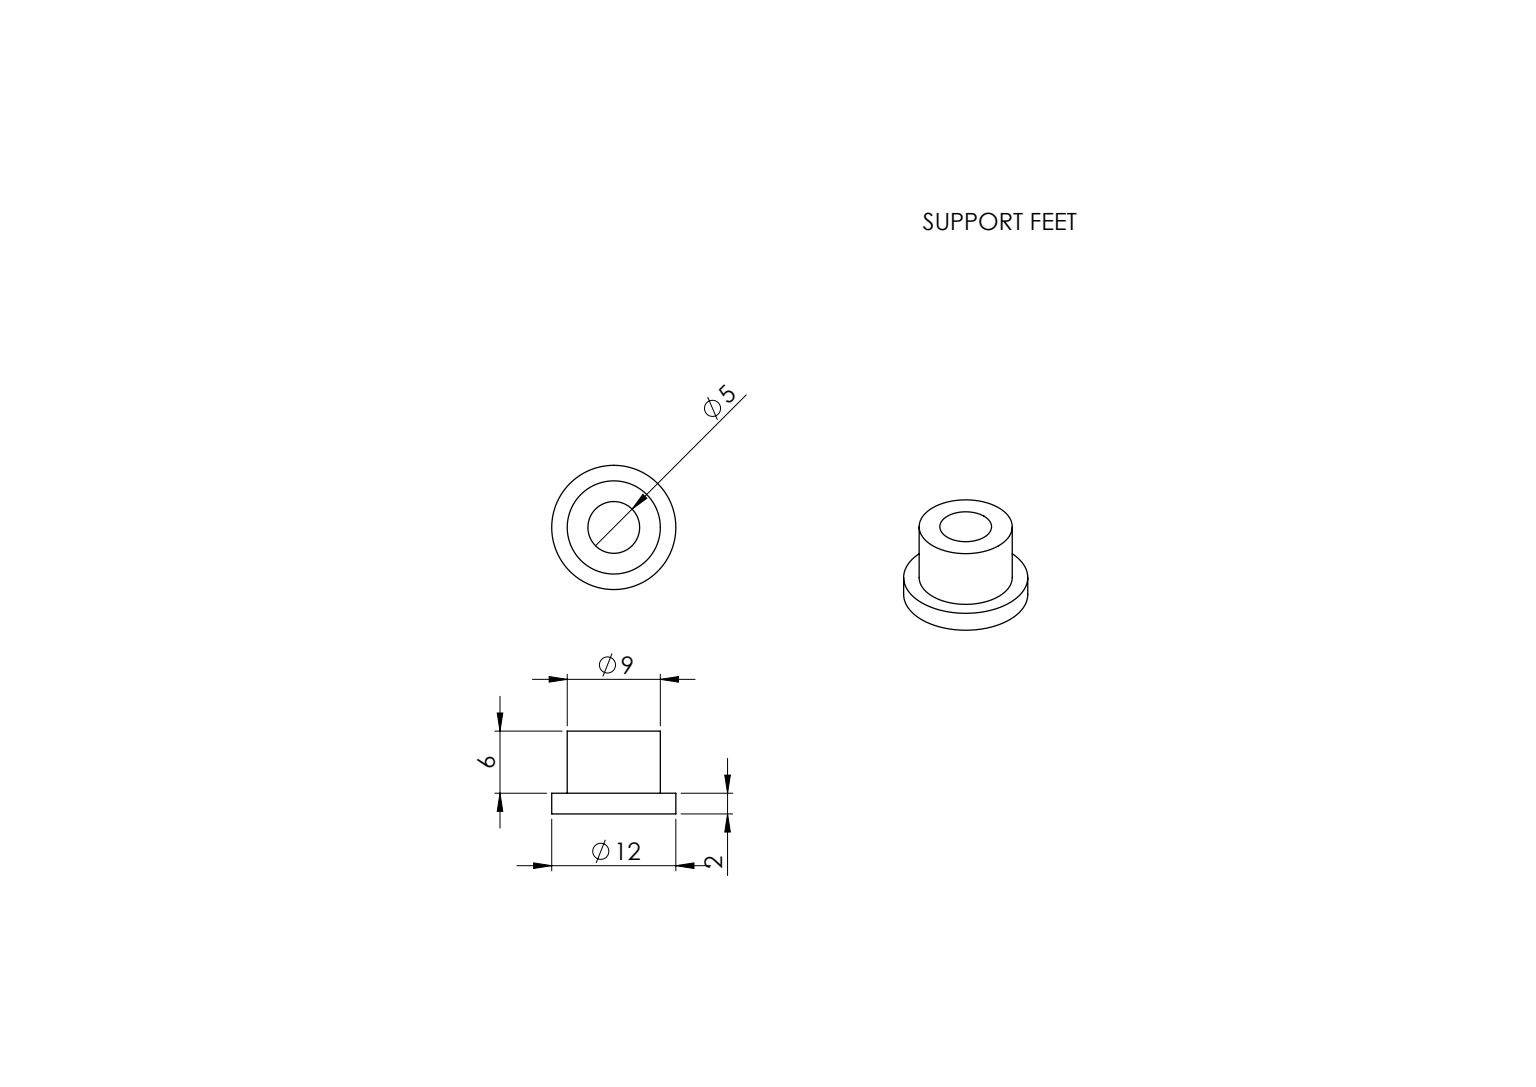
ISO-10303-21;
HEADER;
FILE_DESCRIPTION (('STEP AP214'),
    '1' );
FILE_NAME ('Support Feet^MAS-192.step',
    '2026-10-24T04:45:50',
    ( '' ),
    ( '' ),
    'SwSTEP 2.0',
    'SolidWorks 2026',
    '' );
FILE_SCHEMA (( 'AUTOMOTIVE_DESIGN' ));
ENDSEC;

DATA;
#2=( GEOMETRIC_REPRESENTATION_CONTEXT ( 3 ) GLOBAL_UNCERTAINTY_ASSIGNED_CONTEXT ( ( #2528 ) ) GLOBAL_UNIT_ASSIGNED_CONTEXT ( ( #1633, #2133, #1361 ) ) REPRESENTATION_CONTEXT ( 'NONE', 'WORKASPACE' ) );
#3=DIRECTION ( 'NONE',  ( 0.000000000000000000, -1.000000000000000000, 0.000000000000000000 ) ) ;
#6=ORIENTED_EDGE ( 'NONE', *, *, #1808, .T. ) ;
#13=ORIENTED_EDGE ( 'NONE', *, *, #2082, .F. ) ;
#22=VERTEX_POINT ( 'NONE', #1418 ) ;
#25=PRODUCT ( 'Support Feet^MAS-192', 'Support Feet^MAS-192', '', ( #945 ) ) ;
#74=ORIENTED_EDGE ( 'NONE', *, *, #2863, .T. ) ;
#80=SURFACE_STYLE_USAGE ( .BOTH. , #3231 ) ;
#98=AXIS2_PLACEMENT_3D ( 'NONE', #3255, #906, #600 ) ;
#106=EDGE_CURVE ( 'NONE', #871, #1696, #686, .T. ) ;
#124=ORIENTED_EDGE ( 'NONE', *, *, #674, .T. ) ;
#145=DIRECTION ( 'NONE',  ( -0.000000000000000000, 1.000000000000000000, -0.000000000000000000 ) ) ;
#146=DIRECTION ( 'NONE',  ( 0.000000000000000000, -1.000000000000000000, 0.000000000000000000 ) ) ;
#150=AXIS2_PLACEMENT_3D ( 'NONE', #1095, #3156, #1856 ) ;
#153=MECHANICAL_DESIGN_GEOMETRIC_PRESENTATION_REPRESENTATION('',(#3211),#1787);
#168=ADVANCED_FACE ( 'NONE', ( #219 ), #472, .F. ) ;
#179=SHAPE_REPRESENTATION_RELATIONSHIP ( 'NONE' , 'NONE' ,  #1050, #930 ) ;
#195=EDGE_CURVE ( 'NONE', #2855, #2405, #2542, .T. ) ;
#201=VECTOR ( 'NONE', #2928, 1000.000000000000000 ) ;
#211=DIRECTION ( 'NONE',  ( 0.000000000000000000, -1.000000000000000000, 0.000000000000000000 ) ) ;
#216=( NAMED_UNIT ( * ) PLANE_ANGLE_UNIT ( ) SI_UNIT ( $, .RADIAN. ) );
#219=FACE_OUTER_BOUND ( 'NONE', #3264, .T. ) ;
#222=DIRECTION ( 'NONE',  ( -0.000000000000000000, 1.000000000000000000, -0.000000000000000000 ) ) ;
#245=ORIENTED_EDGE ( 'NONE', *, *, #2920, .T. ) ;
#251=CARTESIAN_POINT ( 'NONE',  ( -66.99999999999997158, -6.000000000000000000, 41.99999999999999289 ) ) ;
#254=ORIENTED_EDGE ( 'NONE', *, *, #2827, .T. ) ;
#261=CARTESIAN_POINT ( 'NONE',  ( -66.99999999999997158, -8.000000000000000000, 41.99999999999999289 ) ) ;
#268=AXIS2_PLACEMENT_3D ( 'NONE', #2067, #1047, #3088 ) ;
#291=CYLINDRICAL_SURFACE ( 'NONE', #701, 4.500000000000010658 ) ;
#322=AXIS2_PLACEMENT_3D ( 'NONE', #1317, #3110, #3142 ) ;
#331=VERTEX_POINT ( 'NONE', #2651 ) ;
#340=ORIENTED_EDGE ( 'NONE', *, *, #1808, .F. ) ;
#348=CARTESIAN_POINT ( 'NONE',  ( -66.99999999999997158, 0.000000000000000000, 46.50000000000000711 ) ) ;
#349=SURFACE_STYLE_FILL_AREA ( #2686 ) ;
#364=( LENGTH_UNIT ( ) NAMED_UNIT ( * ) SI_UNIT ( .MILLI., .METRE. ) );
#370=CIRCLE ( 'NONE', #482, 4.500000000000010658 ) ;
#379=AXIS2_PLACEMENT_3D ( 'NONE', #915, #146, #2518 ) ;
#386=ORIENTED_EDGE ( 'NONE', *, *, #1705, .F. ) ;
#388=DIRECTION ( 'NONE',  ( 0.000000000000000000, 0.000000000000000000, -1.000000000000000000 ) ) ;
#405=CARTESIAN_POINT ( 'NONE',  ( -66.99999999999997158, -8.000000000000000000, 39.49999999999998579 ) ) ;
#415=ORIENTED_EDGE ( 'NONE', *, *, #2685, .T. ) ;
#422=CIRCLE ( 'NONE', #2330, 2.500000000000009326 ) ;
#472=CYLINDRICAL_SURFACE ( 'NONE', #803, 2.500000000000009326 ) ;
#482=AXIS2_PLACEMENT_3D ( 'NONE', #711, #2825, #1752 ) ;
#484=CIRCLE ( 'NONE', #975, 6.000000000000005329 ) ;
#506=EDGE_LOOP ( 'NONE', ( #2297, #1009 ) ) ;
#508=CARTESIAN_POINT ( 'NONE',  ( -66.99999999999997158, -8.000000000000000000, 41.99999999999999289 ) ) ;
#513=EDGE_LOOP ( 'NONE', ( #1170, #1121 ) ) ;
#525=ORIENTED_EDGE ( 'NONE', *, *, #1492, .F. ) ;
#535=EDGE_CURVE ( 'NONE', #871, #3340, #2736, .T. ) ;
#536=AXIS2_PLACEMENT_3D ( 'NONE', #3344, #1291, #2041 ) ;
#547=ORIENTED_EDGE ( 'NONE', *, *, #1705, .T. ) ;
#589=CIRCLE ( 'NONE', #1031, 4.500000000000010658 ) ;
#593=CIRCLE ( 'NONE', #268, 6.000000000000005329 ) ;
#596=ADVANCED_FACE ( 'NONE', ( #3051 ), #1293, .T. ) ;
#600=DIRECTION ( 'NONE',  ( 0.000000000000000000, 0.000000000000000000, -1.000000000000000000 ) ) ;
#606=CARTESIAN_POINT ( 'NONE',  ( -66.99999999999997158, -6.000000000000000000, 44.50000000000000711 ) ) ;
#617=VERTEX_POINT ( 'NONE', #1508 ) ;
#637=AXIS2_PLACEMENT_3D ( 'NONE', #2080, #3362, #966 ) ;
#650=CARTESIAN_POINT ( 'NONE',  ( -66.99999999999997158, 0.000000000000000000, 41.99999999999999289 ) ) ;
#662=CYLINDRICAL_SURFACE ( 'NONE', #1528, 6.000000000000005329 ) ;
#665=DIRECTION ( 'NONE',  ( 0.000000000000000000, -0.000000000000000000, -1.000000000000000000 ) ) ;
#666=EDGE_CURVE ( 'NONE', #617, #22, #2260, .T. ) ;
#674=EDGE_CURVE ( 'NONE', #2405, #2855, #370, .T. ) ;
#681=SHAPE_DEFINITION_REPRESENTATION ( #1034, #1050 ) ;
#686=CIRCLE ( 'NONE', #858, 2.500000000000009326 ) ;
#701=AXIS2_PLACEMENT_3D ( 'NONE', #1590, #222, #1270 ) ;
#711=CARTESIAN_POINT ( 'NONE',  ( -66.99999999999997158, -6.000000000000000000, 41.99999999999999289 ) ) ;
#725=UNCERTAINTY_MEASURE_WITH_UNIT (LENGTH_MEASURE( 1.000000000000000082E-05 ), #364, 'distance_accuracy_value', 'NONE');
#744=DIRECTION ( 'NONE',  ( 0.000000000000000000, -0.000000000000000000, -1.000000000000000000 ) ) ;
#753=FACE_OUTER_BOUND ( 'NONE', #969, .T. ) ;
#760=UNCERTAINTY_MEASURE_WITH_UNIT (LENGTH_MEASURE( 1.000000000000000082E-05 ), #1279, 'distance_accuracy_value', 'NONE');
#767=EDGE_CURVE ( 'NONE', #3340, #1840, #1842, .T. ) ;
#778=ORIENTED_EDGE ( 'NONE', *, *, #535, .T. ) ;
#799=CARTESIAN_POINT ( 'NONE',  ( -66.99999999999997158, -6.000000000000000000, 48.00000000000000000 ) ) ;
#803=AXIS2_PLACEMENT_3D ( 'NONE', #508, #1247, #1756 ) ;
#853=CARTESIAN_POINT ( 'NONE',  ( -66.99999999999997158, -6.000000000000000000, 41.99999999999999289 ) ) ;
#858=AXIS2_PLACEMENT_3D ( 'NONE', #3313, #2011, #3055 ) ;
#871=VERTEX_POINT ( 'NONE', #929 ) ;
#877=EDGE_LOOP ( 'NONE', ( #13, #2657 ) ) ;
#882=PRESENTATION_STYLE_ASSIGNMENT (( #80 ) ) ;
#906=DIRECTION ( 'NONE',  ( 0.000000000000000000, -1.000000000000000000, 0.000000000000000000 ) ) ;
#909=CARTESIAN_POINT ( 'NONE',  ( -66.99999999999997158, 0.000000000000000000, 41.99999999999999289 ) ) ;
#915=CARTESIAN_POINT ( 'NONE',  ( -66.99999999999997158, -6.000000000000000000, 41.99999999999999289 ) ) ;
#925=VECTOR ( 'NONE', #3, 1000.000000000000000 ) ;
#929=CARTESIAN_POINT ( 'NONE',  ( -66.99999999999997158, -6.000000000000000000, 39.49999999999998579 ) ) ;
#930=ADVANCED_BREP_SHAPE_REPRESENTATION ( '', ( #2021, #3111 ), #2 ) ;
#938=CARTESIAN_POINT ( 'NONE',  ( -66.99999999999997158, -8.000000000000000000, 44.50000000000000711 ) ) ;
#945=PRODUCT_CONTEXT ( 'NONE', #1857, 'mechanical' ) ;
#966=DIRECTION ( 'NONE',  ( 0.000000000000000000, 0.000000000000000000, -1.000000000000000000 ) ) ;
#969=EDGE_LOOP ( 'NONE', ( #2568, #3228 ) ) ;
#974=CARTESIAN_POINT ( 'NONE',  ( -66.99999999999997158, -6.000000000000000000, 48.00000000000000000 ) ) ;
#975=AXIS2_PLACEMENT_3D ( 'NONE', #261, #211, #2079 ) ;
#1002=CARTESIAN_POINT ( 'NONE',  ( -66.99999999999997158, -6.000000000000000000, 35.99999999999999289 ) ) ;
#1005=FACE_BOUND ( 'NONE', #506, .T. ) ;
#1009=ORIENTED_EDGE ( 'NONE', *, *, #767, .T. ) ;
#1014=ADVANCED_FACE ( 'NONE', ( #753 ), #1776, .F. ) ;
#1031=AXIS2_PLACEMENT_3D ( 'NONE', #650, #1156, #1434 ) ;
#1034=PRODUCT_DEFINITION_SHAPE ( 'NONE', 'NONE',  #2584 ) ;
#1047=DIRECTION ( 'NONE',  ( 0.000000000000000000, -1.000000000000000000, 0.000000000000000000 ) ) ;
#1050=SHAPE_REPRESENTATION ( 'Support Feet^MAS-192', ( #3111 ), #2 ) ;
#1084=AXIS2_PLACEMENT_3D ( 'NONE', #251, #2301, #2316 ) ;
#1090=AXIS2_PLACEMENT_3D ( 'NONE', #2616, #2119, #3356 ) ;
#1095=CARTESIAN_POINT ( 'NONE',  ( -66.99999999999997158, 0.000000000000000000, 41.99999999999999289 ) ) ;
#1121=ORIENTED_EDGE ( 'NONE', *, *, #1492, .T. ) ;
#1138=ORIENTED_EDGE ( 'NONE', *, *, #1885, .T. ) ;
#1145=AXIS2_PLACEMENT_3D ( 'NONE', #853, #2462, #1878 ) ;
#1156=DIRECTION ( 'NONE',  ( 0.000000000000000000, -1.000000000000000000, 0.000000000000000000 ) ) ;
#1170=ORIENTED_EDGE ( 'NONE', *, *, #2436, .T. ) ;
#1171=ADVANCED_FACE ( 'NONE', ( #2692, #2203 ), #3199, .F. ) ;
#1196=FACE_OUTER_BOUND ( 'NONE', #2237, .T. ) ;
#1208=MECHANICAL_DESIGN_GEOMETRIC_PRESENTATION_REPRESENTATION('',(#1468),#3054);
#1209=ORIENTED_EDGE ( 'NONE', *, *, #666, .T. ) ;
#1215=DIRECTION ( 'NONE',  ( -0.000000000000000000, 1.000000000000000000, -0.000000000000000000 ) ) ;
#1224=ORIENTED_EDGE ( 'NONE', *, *, #2353, .F. ) ;
#1229=CARTESIAN_POINT ( 'NONE',  ( -66.99999999999997158, 0.000000000000000000, 44.50000000000000711 ) ) ;
#1244=CIRCLE ( 'NONE', #379, 2.500000000000009326 ) ;
#1247=DIRECTION ( 'NONE',  ( -0.000000000000000000, 1.000000000000000000, -0.000000000000000000 ) ) ;
#1262=CARTESIAN_POINT ( 'NONE',  ( -66.99999999999997158, -6.000000000000000000, 37.49999999999998579 ) ) ;
#1270=DIRECTION ( 'NONE',  ( 0.000000000000000000, 0.000000000000000000, 1.000000000000000000 ) ) ;
#1279=( LENGTH_UNIT ( ) NAMED_UNIT ( * ) SI_UNIT ( .MILLI., .METRE. ) );
#1291=DIRECTION ( 'NONE',  ( -0.000000000000000000, 1.000000000000000000, -0.000000000000000000 ) ) ;
#1293=CYLINDRICAL_SURFACE ( 'NONE', #637, 6.000000000000005329 ) ;
#1314=CARTESIAN_POINT ( 'NONE',  ( -66.99999999999997158, 0.000000000000000000, 37.49999999999998579 ) ) ;
#1317=CARTESIAN_POINT ( 'NONE',  ( -66.99999999999997158, -8.000000000000000000, 41.99999999999999289 ) ) ;
#1361=( NAMED_UNIT ( * ) SI_UNIT ( $, .STERADIAN. ) SOLID_ANGLE_UNIT ( ) );
#1394=CYLINDRICAL_SURFACE ( 'NONE', #3329, 4.500000000000010658 ) ;
#1418=CARTESIAN_POINT ( 'NONE',  ( -66.99999999999997158, -8.000000000000000000, 35.99999999999999289 ) ) ;
#1432=ORIENTED_EDGE ( 'NONE', *, *, #2774, .F. ) ;
#1434=DIRECTION ( 'NONE',  ( 1.000000000000000000, 0.000000000000000000, 0.000000000000000000 ) ) ;
#1464=VECTOR ( 'NONE', #2850, 1000.000000000000000 ) ;
#1468=STYLED_ITEM ( 'NONE', ( #882 ), #930 ) ;
#1470=COLOUR_RGB ( '',0.8941176470588234615, 0.8941176470588234615, 0.8941176470588234615 ) ;
#1492=EDGE_CURVE ( 'NONE', #331, #22, #2340, .T. ) ;
#1508=CARTESIAN_POINT ( 'NONE',  ( -66.99999999999997158, -6.000000000000000000, 35.99999999999999289 ) ) ;
#1528=AXIS2_PLACEMENT_3D ( 'NONE', #2778, #3031, #2008 ) ;
#1575=CIRCLE ( 'NONE', #2713, 6.000000000000005329 ) ;
#1579=AXIS2_PLACEMENT_3D ( 'NONE', #1963, #2758, #665 ) ;
#1590=CARTESIAN_POINT ( 'NONE',  ( -66.99999999999997158, -8.000000000000000000, 41.99999999999999289 ) ) ;
#1591=EDGE_LOOP ( 'NONE', ( #2711, #1432 ) ) ;
#1603=CARTESIAN_POINT ( 'NONE',  ( -66.99999999999997158, -8.000000000000000000, 41.99999999999999289 ) ) ;
#1633=( LENGTH_UNIT ( ) NAMED_UNIT ( * ) SI_UNIT ( .MILLI., .METRE. ) );
#1696=VERTEX_POINT ( 'NONE', #606 ) ;
#1705=EDGE_CURVE ( 'NONE', #2405, #2003, #2149, .T. ) ;
#1723=PLANE ( 'NONE',  #1579 ) ;
#1752=DIRECTION ( 'NONE',  ( 0.000000000000000000, 0.000000000000000000, -1.000000000000000000 ) ) ;
#1756=DIRECTION ( 'NONE',  ( 0.000000000000000000, 0.000000000000000000, 1.000000000000000000 ) ) ;
#1776=PLANE ( 'NONE',  #1090 ) ;
#1787=( GEOMETRIC_REPRESENTATION_CONTEXT ( 3 ) GLOBAL_UNCERTAINTY_ASSIGNED_CONTEXT ( ( #760 ) ) GLOBAL_UNIT_ASSIGNED_CONTEXT ( ( #1279, #216, #2094 ) ) REPRESENTATION_CONTEXT ( 'NONE', 'WORKASPACE' ) );
#1808=EDGE_CURVE ( 'NONE', #1696, #1840, #1986, .T. ) ;
#1809=CARTESIAN_POINT ( 'NONE',  ( -66.99999999999997158, -6.000000000000000000, 46.50000000000000711 ) ) ;
#1838=VECTOR ( 'NONE', #145, 1000.000000000000000 ) ;
#1840=VERTEX_POINT ( 'NONE', #1229 ) ;
#1842=CIRCLE ( 'NONE', #98, 2.500000000000009326 ) ;
#1856=DIRECTION ( 'NONE',  ( 1.000000000000000000, 0.000000000000000000, 0.000000000000000000 ) ) ;
#1857=APPLICATION_CONTEXT ( 'automotive_design' ) ;
#1861=CARTESIAN_POINT ( 'NONE',  ( -66.99999999999997158, -8.000000000000000000, 46.50000000000000711 ) ) ;
#1871=CARTESIAN_POINT ( 'NONE',  ( 0.000000000000000000, 0.000000000000000000, 0.000000000000000000 ) ) ;
#1878=DIRECTION ( 'NONE',  ( 0.000000000000000000, -0.000000000000000000, -1.000000000000000000 ) ) ;
#1885=EDGE_CURVE ( 'NONE', #1696, #871, #1244, .T. ) ;
#1938=DIRECTION ( 'NONE',  ( 0.000000000000000000, 0.000000000000000000, 1.000000000000000000 ) ) ;
#1963=CARTESIAN_POINT ( 'NONE',  ( -66.99999999999997158, -8.000000000000000000, 41.99999999999999289 ) ) ;
#1978=LINE ( 'NONE', #1861, #1464 ) ;
#1986=LINE ( 'NONE', #938, #3167 ) ;
#1993=CARTESIAN_POINT ( 'NONE',  ( -66.99999999999997158, -6.000000000000000000, 41.99999999999999289 ) ) ;
#2003=VERTEX_POINT ( 'NONE', #1314 ) ;
#2008=DIRECTION ( 'NONE',  ( 0.000000000000000000, 0.000000000000000000, -1.000000000000000000 ) ) ;
#2011=DIRECTION ( 'NONE',  ( 0.000000000000000000, -1.000000000000000000, 0.000000000000000000 ) ) ;
#2014=FACE_OUTER_BOUND ( 'NONE', #513, .T. ) ;
#2021=MANIFOLD_SOLID_BREP ( 'Boss-Extrude1', #2700 ) ;
#2041=DIRECTION ( 'NONE',  ( 0.000000000000000000, 0.000000000000000000, 1.000000000000000000 ) ) ;
#2049=EDGE_LOOP ( 'NONE', ( #2469, #124 ) ) ;
#2057=ORIENTED_EDGE ( 'NONE', *, *, #2082, .T. ) ;
#2067=CARTESIAN_POINT ( 'NONE',  ( -66.99999999999997158, -6.000000000000000000, 41.99999999999999289 ) ) ;
#2079=DIRECTION ( 'NONE',  ( 0.000000000000000000, 0.000000000000000000, -1.000000000000000000 ) ) ;
#2080=CARTESIAN_POINT ( 'NONE',  ( -66.99999999999997158, -6.000000000000000000, 41.99999999999999289 ) ) ;
#2082=EDGE_CURVE ( 'NONE', #2103, #2003, #2988, .T. ) ;
#2094=( NAMED_UNIT ( * ) SI_UNIT ( $, .STERADIAN. ) SOLID_ANGLE_UNIT ( ) );
#2103=VERTEX_POINT ( 'NONE', #348 ) ;
#2117=VECTOR ( 'NONE', #3309, 1000.000000000000000 ) ;
#2119=DIRECTION ( 'NONE',  ( 0.000000000000000000, -1.000000000000000000, 0.000000000000000000 ) ) ;
#2133=( NAMED_UNIT ( * ) PLANE_ANGLE_UNIT ( ) SI_UNIT ( $, .RADIAN. ) );
#2147=FILL_AREA_STYLE_COLOUR ( '', #1470 ) ;
#2149=LINE ( 'NONE', #2383, #201 ) ;
#2150=FACE_OUTER_BOUND ( 'NONE', #2581, .T. ) ;
#2159=ORIENTED_EDGE ( 'NONE', *, *, #535, .F. ) ;
#2203=FACE_OUTER_BOUND ( 'NONE', #1591, .T. ) ;
#2216=DIRECTION ( 'NONE',  ( 0.000000000000000000, 0.000000000000000000, -1.000000000000000000 ) ) ;
#2237=EDGE_LOOP ( 'NONE', ( #74, #245, #2450, #2549 ) ) ;
#2260=LINE ( 'NONE', #1002, #2117 ) ;
#2297=ORIENTED_EDGE ( 'NONE', *, *, #2353, .T. ) ;
#2301=DIRECTION ( 'NONE',  ( 0.000000000000000000, -1.000000000000000000, 0.000000000000000000 ) ) ;
#2316=DIRECTION ( 'NONE',  ( 0.000000000000000000, 0.000000000000000000, -1.000000000000000000 ) ) ;
#2330=AXIS2_PLACEMENT_3D ( 'NONE', #909, #2749, #388 ) ;
#2338=FACE_OUTER_BOUND ( 'NONE', #3118, .T. ) ;
#2340=CIRCLE ( 'NONE', #322, 6.000000000000005329 ) ;
#2349=ORIENTED_EDGE ( 'NONE', *, *, #767, .F. ) ;
#2353=EDGE_CURVE ( 'NONE', #1840, #3340, #422, .T. ) ;
#2354=DIRECTION ( 'NONE',  ( 0.000000000000000000, -1.000000000000000000, 0.000000000000000000 ) ) ;
#2383=CARTESIAN_POINT ( 'NONE',  ( -66.99999999999997158, -8.000000000000000000, 37.49999999999998579 ) ) ;
#2405=VERTEX_POINT ( 'NONE', #1262 ) ;
#2434=DIRECTION ( 'NONE',  ( -0.000000000000000000, 1.000000000000000000, -0.000000000000000000 ) ) ;
#2436=EDGE_CURVE ( 'NONE', #22, #331, #484, .T. ) ;
#2450=ORIENTED_EDGE ( 'NONE', *, *, #2436, .F. ) ;
#2454=( NAMED_UNIT ( * ) PLANE_ANGLE_UNIT ( ) SI_UNIT ( $, .RADIAN. ) );
#2462=DIRECTION ( 'NONE',  ( 0.000000000000000000, -1.000000000000000000, 0.000000000000000000 ) ) ;
#2467=ADVANCED_FACE ( 'NONE', ( #2570 ), #2841, .F. ) ;
#2469=ORIENTED_EDGE ( 'NONE', *, *, #195, .T. ) ;
#2518=DIRECTION ( 'NONE',  ( 0.000000000000000000, 0.000000000000000000, -1.000000000000000000 ) ) ;
#2528=UNCERTAINTY_MEASURE_WITH_UNIT (LENGTH_MEASURE( 1.000000000000000082E-05 ), #1633, 'distance_accuracy_value', 'NONE');
#2542=CIRCLE ( 'NONE', #1084, 4.500000000000010658 ) ;
#2549=ORIENTED_EDGE ( 'NONE', *, *, #666, .F. ) ;
#2568=ORIENTED_EDGE ( 'NONE', *, *, #1885, .F. ) ;
#2570=FACE_OUTER_BOUND ( 'NONE', #3145, .T. ) ;
#2572=PLANE ( 'NONE',  #3278 ) ;
#2581=EDGE_LOOP ( 'NONE', ( #3146, #547, #415, #2890 ) ) ;
#2584=PRODUCT_DEFINITION ( 'UNKNOWN', '', #3229, #3288 ) ;
#2616=CARTESIAN_POINT ( 'NONE',  ( -66.99999999999997158, -6.000000000000000000, 41.99999999999999289 ) ) ;
#2634=ORIENTED_EDGE ( 'NONE', *, *, #106, .T. ) ;
#2639=DIRECTION ( 'NONE',  ( 1.000000000000000000, 0.000000000000000000, 0.000000000000000000 ) ) ;
#2644=EDGE_LOOP ( 'NONE', ( #2744, #3290, #1209, #525 ) ) ;
#2651=CARTESIAN_POINT ( 'NONE',  ( -66.99999999999997158, -8.000000000000000000, 48.00000000000000000 ) ) ;
#2657=ORIENTED_EDGE ( 'NONE', *, *, #2685, .F. ) ;
#2685=EDGE_CURVE ( 'NONE', #2003, #2103, #589, .T. ) ;
#2686=FILL_AREA_STYLE ('',( #2147 ) ) ;
#2692=FACE_BOUND ( 'NONE', #2049, .T. ) ;
#2700=CLOSED_SHELL ( 'NONE', ( #3176, #2467, #2963, #2929, #168, #3292, #1014, #596, #1171, #2791 ) ) ;
#2711=ORIENTED_EDGE ( 'NONE', *, *, #2863, .F. ) ;
#2713=AXIS2_PLACEMENT_3D ( 'NONE', #1993, #3035, #2216 ) ;
#2736=LINE ( 'NONE', #405, #1838 ) ;
#2744=ORIENTED_EDGE ( 'NONE', *, *, #2920, .F. ) ;
#2749=DIRECTION ( 'NONE',  ( 0.000000000000000000, -1.000000000000000000, 0.000000000000000000 ) ) ;
#2758=DIRECTION ( 'NONE',  ( 0.000000000000000000, -1.000000000000000000, 0.000000000000000000 ) ) ;
#2774=EDGE_CURVE ( 'NONE', #2775, #617, #1575, .T. ) ;
#2775=VERTEX_POINT ( 'NONE', #974 ) ;
#2778=CARTESIAN_POINT ( 'NONE',  ( -66.99999999999997158, -6.000000000000000000, 41.99999999999999289 ) ) ;
#2791=ADVANCED_FACE ( 'NONE', ( #2014 ), #1723, .T. ) ;
#2825=DIRECTION ( 'NONE',  ( 0.000000000000000000, -1.000000000000000000, 0.000000000000000000 ) ) ;
#2827=EDGE_CURVE ( 'NONE', #2855, #2103, #1978, .T. ) ;
#2828=FACE_OUTER_BOUND ( 'NONE', #877, .T. ) ;
#2841=CYLINDRICAL_SURFACE ( 'NONE', #536, 2.500000000000009326 ) ;
#2850=DIRECTION ( 'NONE',  ( -0.000000000000000000, 1.000000000000000000, -0.000000000000000000 ) ) ;
#2855=VERTEX_POINT ( 'NONE', #1809 ) ;
#2863=EDGE_CURVE ( 'NONE', #617, #2775, #593, .T. ) ;
#2864=LINE ( 'NONE', #799, #925 ) ;
#2890=ORIENTED_EDGE ( 'NONE', *, *, #2827, .F. ) ;
#2896=( NAMED_UNIT ( * ) SI_UNIT ( $, .STERADIAN. ) SOLID_ANGLE_UNIT ( ) );
#2920=EDGE_CURVE ( 'NONE', #2775, #331, #2864, .T. ) ;
#2921=ORIENTED_EDGE ( 'NONE', *, *, #195, .F. ) ;
#2928=DIRECTION ( 'NONE',  ( -0.000000000000000000, 1.000000000000000000, -0.000000000000000000 ) ) ;
#2929=ADVANCED_FACE ( 'NONE', ( #2338 ), #291, .T. ) ;
#2963=ADVANCED_FACE ( 'NONE', ( #2150 ), #1394, .T. ) ;
#2966=APPLICATION_CONTEXT ( 'automotive_design' ) ;
#2988=CIRCLE ( 'NONE', #150, 4.500000000000010658 ) ;
#3031=DIRECTION ( 'NONE',  ( 0.000000000000000000, -1.000000000000000000, 0.000000000000000000 ) ) ;
#3035=DIRECTION ( 'NONE',  ( 0.000000000000000000, -1.000000000000000000, 0.000000000000000000 ) ) ;
#3051=FACE_OUTER_BOUND ( 'NONE', #2644, .T. ) ;
#3054=( GEOMETRIC_REPRESENTATION_CONTEXT ( 3 ) GLOBAL_UNCERTAINTY_ASSIGNED_CONTEXT ( ( #725 ) ) GLOBAL_UNIT_ASSIGNED_CONTEXT ( ( #364, #2454, #2896 ) ) REPRESENTATION_CONTEXT ( 'NONE', 'WORKASPACE' ) );
#3055=DIRECTION ( 'NONE',  ( 0.000000000000000000, 0.000000000000000000, -1.000000000000000000 ) ) ;
#3088=DIRECTION ( 'NONE',  ( 0.000000000000000000, 0.000000000000000000, -1.000000000000000000 ) ) ;
#3110=DIRECTION ( 'NONE',  ( 0.000000000000000000, -1.000000000000000000, 0.000000000000000000 ) ) ;
#3111=AXIS2_PLACEMENT_3D ( 'NONE', #1871, #3207, #2639 ) ;
#3118=EDGE_LOOP ( 'NONE', ( #386, #2921, #254, #2057 ) ) ;
#3126=CARTESIAN_POINT ( 'NONE',  ( -66.99999999999997158, 0.000000000000000000, 39.49999999999998579 ) ) ;
#3142=DIRECTION ( 'NONE',  ( 0.000000000000000000, 0.000000000000000000, -1.000000000000000000 ) ) ;
#3145=EDGE_LOOP ( 'NONE', ( #1138, #778, #1224, #340 ) ) ;
#3146=ORIENTED_EDGE ( 'NONE', *, *, #674, .F. ) ;
#3156=DIRECTION ( 'NONE',  ( 0.000000000000000000, -1.000000000000000000, 0.000000000000000000 ) ) ;
#3167=VECTOR ( 'NONE', #1215, 1000.000000000000000 ) ;
#3176=ADVANCED_FACE ( 'NONE', ( #1196 ), #662, .T. ) ;
#3199=PLANE ( 'NONE',  #1145 ) ;
#3207=DIRECTION ( 'NONE',  ( 0.000000000000000000, 0.000000000000000000, 1.000000000000000000 ) ) ;
#3211=STYLED_ITEM('',(#3415),#2021);
#3228=ORIENTED_EDGE ( 'NONE', *, *, #106, .F. ) ;
#3229=PRODUCT_DEFINITION_FORMATION_WITH_SPECIFIED_SOURCE ( 'ANY', '', #25, .NOT_KNOWN. ) ;
#3231=SURFACE_SIDE_STYLE ('',( #349 ) ) ;
#3255=CARTESIAN_POINT ( 'NONE',  ( -66.99999999999997158, 0.000000000000000000, 41.99999999999999289 ) ) ;
#3264=EDGE_LOOP ( 'NONE', ( #2159, #2634, #6, #2349 ) ) ;
#3278=AXIS2_PLACEMENT_3D ( 'NONE', #3364, #2354, #744 ) ;
#3288=PRODUCT_DEFINITION_CONTEXT ( 'detailed design', #2966, 'design' ) ;
#3290=ORIENTED_EDGE ( 'NONE', *, *, #2774, .T. ) ;
#3292=ADVANCED_FACE ( 'NONE', ( #2828, #1005 ), #2572, .F. ) ;
#3309=DIRECTION ( 'NONE',  ( 0.000000000000000000, -1.000000000000000000, 0.000000000000000000 ) ) ;
#3313=CARTESIAN_POINT ( 'NONE',  ( -66.99999999999997158, -6.000000000000000000, 41.99999999999999289 ) ) ;
#3329=AXIS2_PLACEMENT_3D ( 'NONE', #1603, #2434, #1938 ) ;
#3340=VERTEX_POINT ( 'NONE', #3126 ) ;
#3344=CARTESIAN_POINT ( 'NONE',  ( -66.99999999999997158, -8.000000000000000000, 41.99999999999999289 ) ) ;
#3356=DIRECTION ( 'NONE',  ( 0.000000000000000000, -0.000000000000000000, -1.000000000000000000 ) ) ;
#3362=DIRECTION ( 'NONE',  ( 0.000000000000000000, -1.000000000000000000, 0.000000000000000000 ) ) ;
#3364=CARTESIAN_POINT ( 'NONE',  ( -66.99999999999997158, 0.000000000000000000, 41.99999999999999289 ) ) ;
#3409=COLOUR_RGB('Grey',0.48,0.52,0.57);
#3410=FILL_AREA_STYLE_COLOUR('',#3409);
#3411=FILL_AREA_STYLE('',(#3410));
#3412=SURFACE_STYLE_FILL_AREA(#3411);
#3413=SURFACE_SIDE_STYLE('',(#3412));
#3414=SURFACE_STYLE_USAGE(.BOTH.,#3413);
#3415=PRESENTATION_STYLE_ASSIGNMENT((#3414));
ENDSEC;
END-ISO-10303-21;
